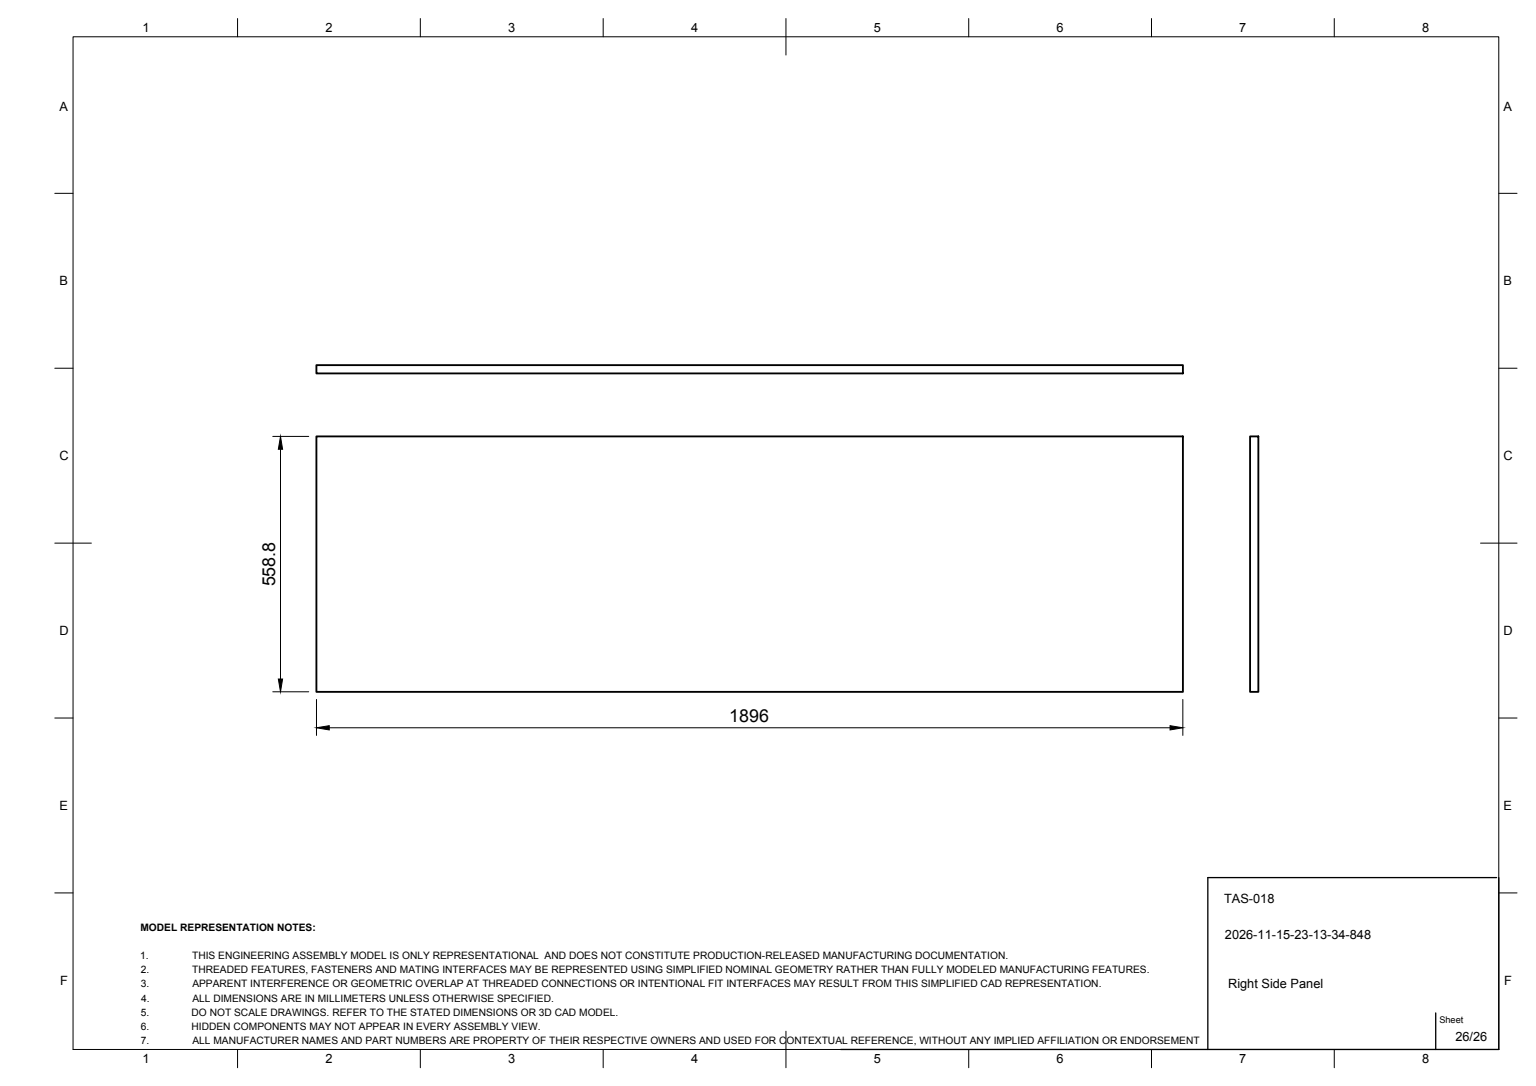
ISO-10303-21;
HEADER;
/* Generated by software containing ST-Developer
 * from STEP Tools, Inc. (www.steptools.com) 
 */

FILE_DESCRIPTION(
/* description */ (''),
/* implementation_level */ '2;1');

FILE_NAME(
/* name */ 'Right Side Panel.step',
/* time_stamp */ '2026-11-15T15:17:57-08:00',
/* author */ (''),
/* organization */ (''),
/* preprocessor_version */ 'ST-DEVELOPER v20.2',
/* originating_system */ 'Autodesk Translation Framework v15.17.0.0',
/* authorisation */ '');

FILE_SCHEMA (('AUTOMOTIVE_DESIGN { 1 0 10303 214 3 1 1 }'));
ENDSEC;

DATA;
#10=MECHANICAL_DESIGN_GEOMETRIC_PRESENTATION_REPRESENTATION('',(#177),#3723);
#129=SHAPE_REPRESENTATION_RELATIONSHIP('SRR','None',#3810,#153);
#153=ADVANCED_BREP_SHAPE_REPRESENTATION('',(#201),#3699);
#177=STYLED_ITEM('',(#3943),#201);
#201=MANIFOLD_SOLID_BREP('Body1',#2025);
#225=FACE_OUTER_BOUND('',#351,.T.);
#226=FACE_OUTER_BOUND('',#352,.T.);
#227=FACE_OUTER_BOUND('',#353,.T.);
#228=FACE_OUTER_BOUND('',#354,.T.);
#229=FACE_OUTER_BOUND('',#355,.T.);
#230=FACE_OUTER_BOUND('',#356,.T.);
#351=EDGE_LOOP('',(#1311,#1312,#1313,#1314));
#352=EDGE_LOOP('',(#1315,#1316,#1317,#1318));
#353=EDGE_LOOP('',(#1319,#1320,#1321,#1322));
#354=EDGE_LOOP('',(#1323,#1324,#1325,#1326));
#355=EDGE_LOOP('',(#1327,#1328,#1329,#1330));
#356=EDGE_LOOP('',(#1331,#1332,#1333,#1334));
#477=LINE('',#3109,#699);
#478=LINE('',#3111,#700);
#479=LINE('',#3113,#701);
#480=LINE('',#3114,#702);
#481=LINE('',#3117,#703);
#482=LINE('',#3119,#704);
#483=LINE('',#3120,#705);
#484=LINE('',#3123,#706);
#485=LINE('',#3125,#707);
#486=LINE('',#3126,#708);
#487=LINE('',#3128,#709);
#488=LINE('',#3129,#710);
#699=VECTOR('',#2511,74.6456692913386);
#700=VECTOR('',#2512,22.);
#701=VECTOR('',#2513,74.6456692913386);
#702=VECTOR('',#2514,22.);
#703=VECTOR('',#2517,0.708661417322833);
#704=VECTOR('',#2518,22.);
#705=VECTOR('',#2519,0.708661417322833);
#706=VECTOR('',#2522,74.6456692913386);
#707=VECTOR('',#2523,22.);
#708=VECTOR('',#2524,74.6456692913386);
#709=VECTOR('',#2527,0.708661417322833);
#710=VECTOR('',#2528,0.708661417322833);
#921=VERTEX_POINT('',#3107);
#922=VERTEX_POINT('',#3108);
#923=VERTEX_POINT('',#3110);
#924=VERTEX_POINT('',#3112);
#925=VERTEX_POINT('',#3116);
#926=VERTEX_POINT('',#3118);
#927=VERTEX_POINT('',#3122);
#928=VERTEX_POINT('',#3124);
#1077=EDGE_CURVE('',#921,#922,#477,.T.);
#1078=EDGE_CURVE('',#923,#922,#478,.T.);
#1079=EDGE_CURVE('',#924,#923,#479,.T.);
#1080=EDGE_CURVE('',#924,#921,#480,.T.);
#1081=EDGE_CURVE('',#922,#925,#481,.T.);
#1082=EDGE_CURVE('',#926,#925,#482,.T.);
#1083=EDGE_CURVE('',#923,#926,#483,.T.);
#1084=EDGE_CURVE('',#925,#927,#484,.T.);
#1085=EDGE_CURVE('',#928,#927,#485,.T.);
#1086=EDGE_CURVE('',#926,#928,#486,.T.);
#1087=EDGE_CURVE('',#927,#921,#487,.T.);
#1088=EDGE_CURVE('',#928,#924,#488,.T.);
#1311=ORIENTED_EDGE('',*,*,#1077,.T.);
#1312=ORIENTED_EDGE('',*,*,#1078,.F.);
#1313=ORIENTED_EDGE('',*,*,#1079,.F.);
#1314=ORIENTED_EDGE('',*,*,#1080,.T.);
#1315=ORIENTED_EDGE('',*,*,#1081,.T.);
#1316=ORIENTED_EDGE('',*,*,#1082,.F.);
#1317=ORIENTED_EDGE('',*,*,#1083,.F.);
#1318=ORIENTED_EDGE('',*,*,#1078,.T.);
#1319=ORIENTED_EDGE('',*,*,#1084,.T.);
#1320=ORIENTED_EDGE('',*,*,#1085,.F.);
#1321=ORIENTED_EDGE('',*,*,#1086,.F.);
#1322=ORIENTED_EDGE('',*,*,#1082,.T.);
#1323=ORIENTED_EDGE('',*,*,#1087,.T.);
#1324=ORIENTED_EDGE('',*,*,#1080,.F.);
#1325=ORIENTED_EDGE('',*,*,#1088,.F.);
#1326=ORIENTED_EDGE('',*,*,#1085,.T.);
#1327=ORIENTED_EDGE('',*,*,#1079,.T.);
#1328=ORIENTED_EDGE('',*,*,#1083,.T.);
#1329=ORIENTED_EDGE('',*,*,#1086,.T.);
#1330=ORIENTED_EDGE('',*,*,#1088,.T.);
#1331=ORIENTED_EDGE('',*,*,#1077,.F.);
#1332=ORIENTED_EDGE('',*,*,#1087,.F.);
#1333=ORIENTED_EDGE('',*,*,#1084,.F.);
#1334=ORIENTED_EDGE('',*,*,#1081,.F.);
#1779=PLANE('',#2317);
#1780=PLANE('',#2318);
#1781=PLANE('',#2319);
#1782=PLANE('',#2320);
#1783=PLANE('',#2321);
#1784=PLANE('',#2322);
#1899=ADVANCED_FACE('',(#225),#1779,.F.);
#1900=ADVANCED_FACE('',(#226),#1780,.F.);
#1901=ADVANCED_FACE('',(#227),#1781,.F.);
#1902=ADVANCED_FACE('',(#228),#1782,.F.);
#1903=ADVANCED_FACE('',(#229),#1783,.F.);
#1904=ADVANCED_FACE('',(#230),#1784,.T.);
#2025=CLOSED_SHELL('',(#1899,#1900,#1901,#1902,#1903,#1904));
#2316=AXIS2_PLACEMENT_3D('',#3105,#2507,#2508);
#2317=AXIS2_PLACEMENT_3D('',#3106,#2509,#2510);
#2318=AXIS2_PLACEMENT_3D('',#3115,#2515,#2516);
#2319=AXIS2_PLACEMENT_3D('',#3121,#2520,#2521);
#2320=AXIS2_PLACEMENT_3D('',#3127,#2525,#2526);
#2321=AXIS2_PLACEMENT_3D('',#3130,#2529,#2530);
#2322=AXIS2_PLACEMENT_3D('',#3131,#2531,#2532);
#2507=DIRECTION('axis',(0.,0.,1.));
#2508=DIRECTION('refdir',(1.,0.,0.));
#2509=DIRECTION('center_axis',(-1.,-1.17112133399278E-16,0.));
#2510=DIRECTION('ref_axis',(0.,0.,1.));
#2511=DIRECTION('',(-1.49903530751076E-16,1.,0.));
#2512=DIRECTION('',(0.,0.,-1.));
#2513=DIRECTION('',(-1.49903530751076E-16,1.,0.));
#2514=DIRECTION('',(0.,0.,-1.));
#2515=DIRECTION('center_axis',(0.,-1.,0.));
#2516=DIRECTION('ref_axis',(0.,0.,-1.));
#2517=DIRECTION('',(-1.,0.,0.));
#2518=DIRECTION('',(0.,0.,-1.));
#2519=DIRECTION('',(-1.,0.,0.));
#2520=DIRECTION('center_axis',(1.,1.17112133399278E-16,0.));
#2521=DIRECTION('ref_axis',(0.,0.,-1.));
#2522=DIRECTION('',(1.49903530751076E-16,-1.,0.));
#2523=DIRECTION('',(0.,0.,-1.));
#2524=DIRECTION('',(1.49903530751076E-16,-1.,0.));
#2525=DIRECTION('center_axis',(0.,1.,0.));
#2526=DIRECTION('ref_axis',(0.,0.,1.));
#2527=DIRECTION('',(1.,0.,0.));
#2528=DIRECTION('',(1.,0.,0.));
#2529=DIRECTION('center_axis',(0.,0.,-1.));
#2530=DIRECTION('ref_axis',(-1.,0.,0.));
#2531=DIRECTION('center_axis',(0.,0.,-1.));
#2532=DIRECTION('ref_axis',(-1.,0.,0.));
#3105=CARTESIAN_POINT('',(0.,0.,0.));
#3106=CARTESIAN_POINT('Origin',(36.,79.2913385826772,22.));
#3107=CARTESIAN_POINT('',(36.,4.64566929133859,0.));
#3108=CARTESIAN_POINT('',(36.,79.2913385826772,0.));
#3109=CARTESIAN_POINT('',(36.,4.64566929133859,0.));
#3110=CARTESIAN_POINT('',(36.,79.2913385826772,22.));
#3111=CARTESIAN_POINT('',(36.,79.2913385826772,22.));
#3112=CARTESIAN_POINT('',(36.,4.64566929133859,22.));
#3113=CARTESIAN_POINT('',(36.,4.64566929133859,22.));
#3114=CARTESIAN_POINT('',(36.,4.64566929133859,22.));
#3115=CARTESIAN_POINT('Origin',(36.,79.2913385826772,22.));
#3116=CARTESIAN_POINT('',(35.2913385826772,79.2913385826772,0.));
#3117=CARTESIAN_POINT('',(36.,79.2913385826772,0.));
#3118=CARTESIAN_POINT('',(35.2913385826772,79.2913385826772,22.));
#3119=CARTESIAN_POINT('',(35.2913385826772,79.2913385826772,22.));
#3120=CARTESIAN_POINT('',(36.,79.2913385826772,22.));
#3121=CARTESIAN_POINT('Origin',(35.2913385826772,79.2913385826772,22.));
#3122=CARTESIAN_POINT('',(35.2913385826772,4.64566929133859,0.));
#3123=CARTESIAN_POINT('',(35.2913385826772,79.2913385826772,0.));
#3124=CARTESIAN_POINT('',(35.2913385826772,4.64566929133859,22.));
#3125=CARTESIAN_POINT('',(35.2913385826772,4.64566929133859,22.));
#3126=CARTESIAN_POINT('',(35.2913385826772,79.2913385826772,22.));
#3127=CARTESIAN_POINT('Origin',(36.,4.64566929133859,22.));
#3128=CARTESIAN_POINT('',(35.2913385826772,4.64566929133859,0.));
#3129=CARTESIAN_POINT('',(35.2913385826772,4.64566929133859,22.));
#3130=CARTESIAN_POINT('Origin',(0.,0.,22.));
#3131=CARTESIAN_POINT('Origin',(0.,0.,0.));
#3672=UNCERTAINTY_MEASURE_WITH_UNIT(LENGTH_MEASURE(0.000393700787401575),
#3725,'DISTANCE_ACCURACY_VALUE',
'Maximum model space distance between geometric entities at asserted c
onnectivities');
#3696=UNCERTAINTY_MEASURE_WITH_UNIT(LENGTH_MEASURE(0.000393700787401575),
#3725,'DISTANCE_ACCURACY_VALUE',
'Maximum model space distance between geometric entities at asserted c
onnectivities');
#3699=(
GEOMETRIC_REPRESENTATION_CONTEXT(3)
GLOBAL_UNCERTAINTY_ASSIGNED_CONTEXT((#3672))
GLOBAL_UNIT_ASSIGNED_CONTEXT((#3725,#3729,#3730))
REPRESENTATION_CONTEXT('','3D')
);
#3723=(
GEOMETRIC_REPRESENTATION_CONTEXT(3)
GLOBAL_UNCERTAINTY_ASSIGNED_CONTEXT((#3696))
GLOBAL_UNIT_ASSIGNED_CONTEXT((#3725,#3729,#3730))
REPRESENTATION_CONTEXT('','3D')
);
#3724=DIMENSIONAL_EXPONENTS(1.,0.,0.,0.,0.,0.,0.);
#3725=(
CONVERSION_BASED_UNIT('inch',#3728)
LENGTH_UNIT()
NAMED_UNIT(#3724)
);
#3726=(
LENGTH_UNIT()
NAMED_UNIT(*)
SI_UNIT(.MILLI.,.METRE.)
);
#3728=LENGTH_MEASURE_WITH_UNIT(LENGTH_MEASURE(25.4),#3726);
#3729=(
NAMED_UNIT(*)
PLANE_ANGLE_UNIT()
SI_UNIT($,.RADIAN.)
);
#3730=(
NAMED_UNIT(*)
SI_UNIT($,.STERADIAN.)
SOLID_ANGLE_UNIT()
);
#3733=SHAPE_DEFINITION_REPRESENTATION(#3759,#3810);
#3759=PRODUCT_DEFINITION_SHAPE('',$,#3837);
#3810=SHAPE_REPRESENTATION('',(#2316),#3699);
#3834=PRODUCT_DEFINITION_CONTEXT('part definition',#3914,'design');
#3837=PRODUCT_DEFINITION('2026-11-15-23-13-34-848','Right Side Panel',#3863,
#3834);
#3863=PRODUCT_DEFINITION_FORMATION('',$,#3918);
#3914=APPLICATION_CONTEXT(
'Core Data for Automotive Mechanical Design Process');
#3915=PRODUCT_CONTEXT('part definition',#3914,'mechanical');
#3918=PRODUCT('2026-11-15-23-13-34-848','Right Side Panel',$,(#3915));
#3943=PRESENTATION_STYLE_ASSIGNMENT((#3951));
#3951=SURFACE_STYLE_USAGE(.BOTH.,#3959);
#3959=SURFACE_SIDE_STYLE('',(#3967));
#3967=SURFACE_STYLE_FILL_AREA(#3975);
#3975=FILL_AREA_STYLE('Dark Blue',(#3983));
#3983=FILL_AREA_STYLE_COLOUR('Dark Blue',#3991);
#3991=COLOUR_RGB('Dark Blue',0.,0.125490196078431,0.376470588235294);
ENDSEC;
END-ISO-10303-21;
